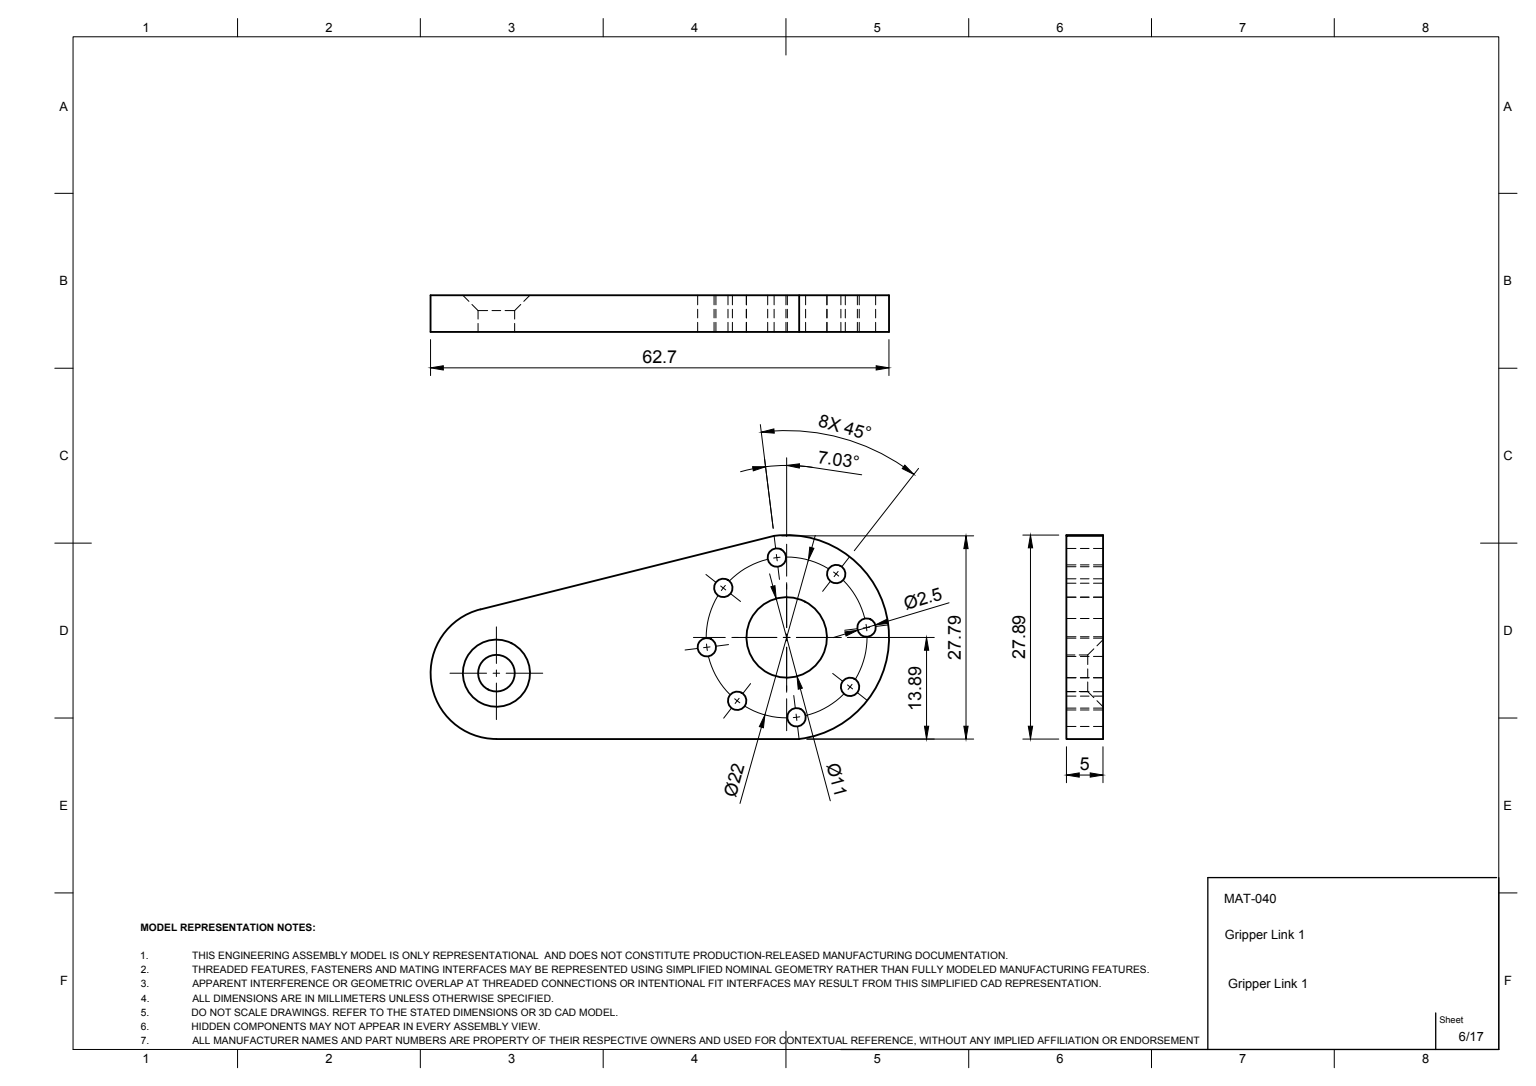
ISO-10303-21;
HEADER;
/* Generated by software containing ST-Developer
 * from STEP Tools, Inc. (www.steptools.com) 
 */

FILE_DESCRIPTION(
/* description */ ('STEP AP214'),
/* implementation_level */ '2;1');

FILE_NAME(
/* name */ 'Gripper Link 1.step',
/* time_stamp */ '2026-11-14T21:53:28-08:00',
/* author */ (''),
/* organization */ (''),
/* preprocessor_version */ 'ST-DEVELOPER v20.2',
/* originating_system */ 'Autodesk Translation Framework v15.17.0.0',
/* authorisation */ '');

FILE_SCHEMA (('AUTOMOTIVE_DESIGN { 1 0 10303 214 3 1 1 }'));
ENDSEC;

DATA;
#10=MECHANICAL_DESIGN_GEOMETRIC_PRESENTATION_REPRESENTATION('',(#329),#20176);
#214=CONICAL_SURFACE('',#11867,4.59,0.785398163397449);
#297=SHAPE_REPRESENTATION_RELATIONSHIP('SRR','None',#20259,#309);
#309=ADVANCED_BREP_SHAPE_REPRESENTATION('',(#356),#20165);
#329=STYLED_ITEM('',(#20337),#356);
#356=MANIFOLD_SOLID_BREP('Body1',#10947);
#516=FACE_BOUND('',#2077,.T.);
#517=FACE_BOUND('',#2078,.T.);
#518=FACE_BOUND('',#2079,.T.);
#519=FACE_BOUND('',#2080,.T.);
#520=FACE_BOUND('',#2081,.T.);
#521=FACE_BOUND('',#2082,.T.);
#522=FACE_BOUND('',#2083,.T.);
#523=FACE_BOUND('',#2084,.T.);
#524=FACE_BOUND('',#2085,.T.);
#525=FACE_BOUND('',#2086,.T.);
#526=FACE_BOUND('',#2088,.T.);
#527=FACE_BOUND('',#2089,.T.);
#528=FACE_BOUND('',#2090,.T.);
#529=FACE_BOUND('',#2091,.T.);
#530=FACE_BOUND('',#2092,.T.);
#531=FACE_BOUND('',#2093,.T.);
#532=FACE_BOUND('',#2094,.T.);
#533=FACE_BOUND('',#2095,.T.);
#534=FACE_BOUND('',#2096,.T.);
#535=FACE_BOUND('',#2097,.T.);
#822=PLANE('',#11900);
#823=PLANE('',#11903);
#824=PLANE('',#11908);
#825=PLANE('',#11909);
#1337=FACE_OUTER_BOUND('',#2065,.T.);
#1338=FACE_OUTER_BOUND('',#2066,.T.);
#1339=FACE_OUTER_BOUND('',#2067,.T.);
#1340=FACE_OUTER_BOUND('',#2068,.T.);
#1341=FACE_OUTER_BOUND('',#2069,.T.);
#1342=FACE_OUTER_BOUND('',#2070,.T.);
#1343=FACE_OUTER_BOUND('',#2071,.T.);
#1344=FACE_OUTER_BOUND('',#2072,.T.);
#1345=FACE_OUTER_BOUND('',#2073,.T.);
#1346=FACE_OUTER_BOUND('',#2074,.T.);
#1347=FACE_OUTER_BOUND('',#2075,.T.);
#1348=FACE_OUTER_BOUND('',#2076,.T.);
#1349=FACE_OUTER_BOUND('',#2087,.T.);
#1350=FACE_OUTER_BOUND('',#2098,.T.);
#1351=FACE_OUTER_BOUND('',#2099,.T.);
#1352=FACE_OUTER_BOUND('',#2100,.T.);
#1353=FACE_OUTER_BOUND('',#2101,.T.);
#2065=EDGE_LOOP('',(#9471,#9472,#9473,#9474,#9475));
#2066=EDGE_LOOP('',(#9476,#9477,#9478,#9479));
#2067=EDGE_LOOP('',(#9480,#9481,#9482,#9483));
#2068=EDGE_LOOP('',(#9484,#9485,#9486,#9487));
#2069=EDGE_LOOP('',(#9488,#9489,#9490,#9491));
#2070=EDGE_LOOP('',(#9492,#9493,#9494,#9495));
#2071=EDGE_LOOP('',(#9496,#9497,#9498,#9499));
#2072=EDGE_LOOP('',(#9500,#9501,#9502,#9503));
#2073=EDGE_LOOP('',(#9504,#9505,#9506,#9507));
#2074=EDGE_LOOP('',(#9508,#9509,#9510,#9511));
#2075=EDGE_LOOP('',(#9512,#9513,#9514,#9515,#9516));
#2076=EDGE_LOOP('',(#9517,#9518,#9519,#9520));
#2077=EDGE_LOOP('',(#9521));
#2078=EDGE_LOOP('',(#9522));
#2079=EDGE_LOOP('',(#9523));
#2080=EDGE_LOOP('',(#9524));
#2081=EDGE_LOOP('',(#9525));
#2082=EDGE_LOOP('',(#9526));
#2083=EDGE_LOOP('',(#9527));
#2084=EDGE_LOOP('',(#9528));
#2085=EDGE_LOOP('',(#9529));
#2086=EDGE_LOOP('',(#9530));
#2087=EDGE_LOOP('',(#9531,#9532,#9533,#9534));
#2088=EDGE_LOOP('',(#9535));
#2089=EDGE_LOOP('',(#9536));
#2090=EDGE_LOOP('',(#9537));
#2091=EDGE_LOOP('',(#9538));
#2092=EDGE_LOOP('',(#9539));
#2093=EDGE_LOOP('',(#9540));
#2094=EDGE_LOOP('',(#9541));
#2095=EDGE_LOOP('',(#9542));
#2096=EDGE_LOOP('',(#9543));
#2097=EDGE_LOOP('',(#9544));
#2098=EDGE_LOOP('',(#9545,#9546,#9547,#9548));
#2099=EDGE_LOOP('',(#9549,#9550,#9551,#9552));
#2100=EDGE_LOOP('',(#9553,#9554,#9555,#9556));
#2101=EDGE_LOOP('',(#9557,#9558,#9559,#9560));
#3069=LINE('',#19370,#4057);
#3070=LINE('',#19377,#4058);
#3071=LINE('',#19383,#4059);
#3072=LINE('',#19389,#4060);
#3073=LINE('',#19395,#4061);
#3074=LINE('',#19401,#4062);
#3075=LINE('',#19407,#4063);
#3076=LINE('',#19413,#4064);
#3077=LINE('',#19419,#4065);
#3078=LINE('',#19425,#4066);
#3079=LINE('',#19429,#4067);
#3080=LINE('',#19434,#4068);
#3081=LINE('',#19438,#4069);
#3082=LINE('',#19445,#4070);
#3083=LINE('',#19448,#4071);
#3084=LINE('',#19450,#4072);
#3085=LINE('',#19451,#4073);
#3086=LINE('',#19453,#4074);
#3087=LINE('',#19454,#4075);
#4057=VECTOR('',#14533,4.59);
#4058=VECTOR('',#14542,1.25);
#4059=VECTOR('',#14549,1.25);
#4060=VECTOR('',#14556,1.25);
#4061=VECTOR('',#14563,1.25);
#4062=VECTOR('',#14570,1.25);
#4063=VECTOR('',#14577,1.25);
#4064=VECTOR('',#14584,1.25);
#4065=VECTOR('',#14591,1.25);
#4066=VECTOR('',#14598,5.5);
#4067=VECTOR('',#14603,2.5);
#4068=VECTOR('',#14608,1000.);
#4069=VECTOR('',#14611,1000.);
#4070=VECTOR('',#14618,1000.);
#4071=VECTOR('',#14621,1000.);
#4072=VECTOR('',#14624,1000.);
#4073=VECTOR('',#14625,1000.);
#4074=VECTOR('',#14628,1000.);
#4075=VECTOR('',#14629,1000.);
#4589=CIRCLE('',#11868,2.5);
#4590=CIRCLE('',#11869,4.59);
#4591=CIRCLE('',#11870,2.5);
#4592=CIRCLE('',#11872,1.25);
#4593=CIRCLE('',#11873,1.25);
#4594=CIRCLE('',#11875,1.25);
#4595=CIRCLE('',#11876,1.25);
#4596=CIRCLE('',#11878,1.25);
#4597=CIRCLE('',#11879,1.25);
#4598=CIRCLE('',#11881,1.25);
#4599=CIRCLE('',#11882,1.25);
#4600=CIRCLE('',#11884,1.25);
#4601=CIRCLE('',#11885,1.25);
#4602=CIRCLE('',#11887,1.25);
#4603=CIRCLE('',#11888,1.25);
#4604=CIRCLE('',#11890,1.25);
#4605=CIRCLE('',#11891,1.25);
#4606=CIRCLE('',#11893,1.25);
#4607=CIRCLE('',#11894,1.25);
#4608=CIRCLE('',#11896,5.5);
#4609=CIRCLE('',#11897,5.5);
#4610=CIRCLE('',#11899,2.5);
#4611=CIRCLE('',#11901,14.);
#4612=CIRCLE('',#11902,9.);
#4613=CIRCLE('',#11904,14.);
#4614=CIRCLE('',#11905,9.);
#5460=VERTEX_POINT('',#19366);
#5461=VERTEX_POINT('',#19367);
#5462=VERTEX_POINT('',#19369);
#5463=VERTEX_POINT('',#19374);
#5464=VERTEX_POINT('',#19376);
#5465=VERTEX_POINT('',#19380);
#5466=VERTEX_POINT('',#19382);
#5467=VERTEX_POINT('',#19386);
#5468=VERTEX_POINT('',#19388);
#5469=VERTEX_POINT('',#19392);
#5470=VERTEX_POINT('',#19394);
#5471=VERTEX_POINT('',#19398);
#5472=VERTEX_POINT('',#19400);
#5473=VERTEX_POINT('',#19404);
#5474=VERTEX_POINT('',#19406);
#5475=VERTEX_POINT('',#19410);
#5476=VERTEX_POINT('',#19412);
#5477=VERTEX_POINT('',#19416);
#5478=VERTEX_POINT('',#19418);
#5479=VERTEX_POINT('',#19422);
#5480=VERTEX_POINT('',#19424);
#5481=VERTEX_POINT('',#19428);
#5482=VERTEX_POINT('',#19432);
#5483=VERTEX_POINT('',#19433);
#5484=VERTEX_POINT('',#19435);
#5485=VERTEX_POINT('',#19437);
#5486=VERTEX_POINT('',#19441);
#5487=VERTEX_POINT('',#19442);
#5488=VERTEX_POINT('',#19444);
#5489=VERTEX_POINT('',#19446);
#6846=EDGE_CURVE('',#5460,#5461,#4589,.T.);
#6847=EDGE_CURVE('',#5461,#5462,#3069,.T.);
#6848=EDGE_CURVE('',#5462,#5462,#4590,.T.);
#6849=EDGE_CURVE('',#5461,#5460,#4591,.T.);
#6850=EDGE_CURVE('',#5463,#5463,#4592,.T.);
#6851=EDGE_CURVE('',#5463,#5464,#3070,.T.);
#6852=EDGE_CURVE('',#5464,#5464,#4593,.T.);
#6853=EDGE_CURVE('',#5465,#5465,#4594,.T.);
#6854=EDGE_CURVE('',#5465,#5466,#3071,.T.);
#6855=EDGE_CURVE('',#5466,#5466,#4595,.T.);
#6856=EDGE_CURVE('',#5467,#5467,#4596,.T.);
#6857=EDGE_CURVE('',#5467,#5468,#3072,.T.);
#6858=EDGE_CURVE('',#5468,#5468,#4597,.T.);
#6859=EDGE_CURVE('',#5469,#5469,#4598,.T.);
#6860=EDGE_CURVE('',#5469,#5470,#3073,.T.);
#6861=EDGE_CURVE('',#5470,#5470,#4599,.T.);
#6862=EDGE_CURVE('',#5471,#5471,#4600,.T.);
#6863=EDGE_CURVE('',#5471,#5472,#3074,.T.);
#6864=EDGE_CURVE('',#5472,#5472,#4601,.T.);
#6865=EDGE_CURVE('',#5473,#5473,#4602,.T.);
#6866=EDGE_CURVE('',#5473,#5474,#3075,.T.);
#6867=EDGE_CURVE('',#5474,#5474,#4603,.T.);
#6868=EDGE_CURVE('',#5475,#5475,#4604,.T.);
#6869=EDGE_CURVE('',#5475,#5476,#3076,.T.);
#6870=EDGE_CURVE('',#5476,#5476,#4605,.T.);
#6871=EDGE_CURVE('',#5477,#5477,#4606,.T.);
#6872=EDGE_CURVE('',#5477,#5478,#3077,.T.);
#6873=EDGE_CURVE('',#5478,#5478,#4607,.T.);
#6874=EDGE_CURVE('',#5479,#5479,#4608,.T.);
#6875=EDGE_CURVE('',#5479,#5480,#3078,.T.);
#6876=EDGE_CURVE('',#5480,#5480,#4609,.T.);
#6877=EDGE_CURVE('',#5460,#5481,#3079,.T.);
#6878=EDGE_CURVE('',#5481,#5481,#4610,.T.);
#6879=EDGE_CURVE('',#5482,#5483,#3080,.T.);
#6880=EDGE_CURVE('',#5482,#5484,#4611,.T.);
#6881=EDGE_CURVE('',#5484,#5485,#3081,.T.);
#6882=EDGE_CURVE('',#5485,#5483,#4612,.T.);
#6883=EDGE_CURVE('',#5486,#5487,#4613,.T.);
#6884=EDGE_CURVE('',#5486,#5488,#3082,.T.);
#6885=EDGE_CURVE('',#5489,#5488,#4614,.T.);
#6886=EDGE_CURVE('',#5487,#5489,#3083,.T.);
#6887=EDGE_CURVE('',#5484,#5487,#3084,.T.);
#6888=EDGE_CURVE('',#5482,#5486,#3085,.T.);
#6889=EDGE_CURVE('',#5489,#5485,#3086,.T.);
#6890=EDGE_CURVE('',#5488,#5483,#3087,.T.);
#9471=ORIENTED_EDGE('',*,*,#6846,.T.);
#9472=ORIENTED_EDGE('',*,*,#6847,.T.);
#9473=ORIENTED_EDGE('',*,*,#6848,.T.);
#9474=ORIENTED_EDGE('',*,*,#6847,.F.);
#9475=ORIENTED_EDGE('',*,*,#6849,.T.);
#9476=ORIENTED_EDGE('',*,*,#6850,.F.);
#9477=ORIENTED_EDGE('',*,*,#6851,.T.);
#9478=ORIENTED_EDGE('',*,*,#6852,.T.);
#9479=ORIENTED_EDGE('',*,*,#6851,.F.);
#9480=ORIENTED_EDGE('',*,*,#6853,.F.);
#9481=ORIENTED_EDGE('',*,*,#6854,.T.);
#9482=ORIENTED_EDGE('',*,*,#6855,.T.);
#9483=ORIENTED_EDGE('',*,*,#6854,.F.);
#9484=ORIENTED_EDGE('',*,*,#6856,.F.);
#9485=ORIENTED_EDGE('',*,*,#6857,.T.);
#9486=ORIENTED_EDGE('',*,*,#6858,.T.);
#9487=ORIENTED_EDGE('',*,*,#6857,.F.);
#9488=ORIENTED_EDGE('',*,*,#6859,.F.);
#9489=ORIENTED_EDGE('',*,*,#6860,.T.);
#9490=ORIENTED_EDGE('',*,*,#6861,.T.);
#9491=ORIENTED_EDGE('',*,*,#6860,.F.);
#9492=ORIENTED_EDGE('',*,*,#6862,.F.);
#9493=ORIENTED_EDGE('',*,*,#6863,.T.);
#9494=ORIENTED_EDGE('',*,*,#6864,.T.);
#9495=ORIENTED_EDGE('',*,*,#6863,.F.);
#9496=ORIENTED_EDGE('',*,*,#6865,.F.);
#9497=ORIENTED_EDGE('',*,*,#6866,.T.);
#9498=ORIENTED_EDGE('',*,*,#6867,.T.);
#9499=ORIENTED_EDGE('',*,*,#6866,.F.);
#9500=ORIENTED_EDGE('',*,*,#6868,.F.);
#9501=ORIENTED_EDGE('',*,*,#6869,.T.);
#9502=ORIENTED_EDGE('',*,*,#6870,.T.);
#9503=ORIENTED_EDGE('',*,*,#6869,.F.);
#9504=ORIENTED_EDGE('',*,*,#6871,.F.);
#9505=ORIENTED_EDGE('',*,*,#6872,.T.);
#9506=ORIENTED_EDGE('',*,*,#6873,.T.);
#9507=ORIENTED_EDGE('',*,*,#6872,.F.);
#9508=ORIENTED_EDGE('',*,*,#6874,.T.);
#9509=ORIENTED_EDGE('',*,*,#6875,.T.);
#9510=ORIENTED_EDGE('',*,*,#6876,.F.);
#9511=ORIENTED_EDGE('',*,*,#6875,.F.);
#9512=ORIENTED_EDGE('',*,*,#6846,.F.);
#9513=ORIENTED_EDGE('',*,*,#6877,.T.);
#9514=ORIENTED_EDGE('',*,*,#6878,.F.);
#9515=ORIENTED_EDGE('',*,*,#6877,.F.);
#9516=ORIENTED_EDGE('',*,*,#6849,.F.);
#9517=ORIENTED_EDGE('',*,*,#6879,.F.);
#9518=ORIENTED_EDGE('',*,*,#6880,.T.);
#9519=ORIENTED_EDGE('',*,*,#6881,.T.);
#9520=ORIENTED_EDGE('',*,*,#6882,.T.);
#9521=ORIENTED_EDGE('',*,*,#6852,.F.);
#9522=ORIENTED_EDGE('',*,*,#6855,.F.);
#9523=ORIENTED_EDGE('',*,*,#6858,.F.);
#9524=ORIENTED_EDGE('',*,*,#6861,.F.);
#9525=ORIENTED_EDGE('',*,*,#6864,.F.);
#9526=ORIENTED_EDGE('',*,*,#6867,.F.);
#9527=ORIENTED_EDGE('',*,*,#6870,.F.);
#9528=ORIENTED_EDGE('',*,*,#6873,.F.);
#9529=ORIENTED_EDGE('',*,*,#6874,.F.);
#9530=ORIENTED_EDGE('',*,*,#6848,.F.);
#9531=ORIENTED_EDGE('',*,*,#6883,.F.);
#9532=ORIENTED_EDGE('',*,*,#6884,.T.);
#9533=ORIENTED_EDGE('',*,*,#6885,.F.);
#9534=ORIENTED_EDGE('',*,*,#6886,.F.);
#9535=ORIENTED_EDGE('',*,*,#6876,.T.);
#9536=ORIENTED_EDGE('',*,*,#6850,.T.);
#9537=ORIENTED_EDGE('',*,*,#6853,.T.);
#9538=ORIENTED_EDGE('',*,*,#6856,.T.);
#9539=ORIENTED_EDGE('',*,*,#6859,.T.);
#9540=ORIENTED_EDGE('',*,*,#6862,.T.);
#9541=ORIENTED_EDGE('',*,*,#6865,.T.);
#9542=ORIENTED_EDGE('',*,*,#6868,.T.);
#9543=ORIENTED_EDGE('',*,*,#6871,.T.);
#9544=ORIENTED_EDGE('',*,*,#6878,.T.);
#9545=ORIENTED_EDGE('',*,*,#6883,.T.);
#9546=ORIENTED_EDGE('',*,*,#6887,.F.);
#9547=ORIENTED_EDGE('',*,*,#6880,.F.);
#9548=ORIENTED_EDGE('',*,*,#6888,.T.);
#9549=ORIENTED_EDGE('',*,*,#6882,.F.);
#9550=ORIENTED_EDGE('',*,*,#6889,.F.);
#9551=ORIENTED_EDGE('',*,*,#6885,.T.);
#9552=ORIENTED_EDGE('',*,*,#6890,.T.);
#9553=ORIENTED_EDGE('',*,*,#6879,.T.);
#9554=ORIENTED_EDGE('',*,*,#6890,.F.);
#9555=ORIENTED_EDGE('',*,*,#6884,.F.);
#9556=ORIENTED_EDGE('',*,*,#6888,.F.);
#9557=ORIENTED_EDGE('',*,*,#6881,.F.);
#9558=ORIENTED_EDGE('',*,*,#6887,.T.);
#9559=ORIENTED_EDGE('',*,*,#6886,.T.);
#9560=ORIENTED_EDGE('',*,*,#6889,.T.);
#10299=CYLINDRICAL_SURFACE('',#11871,1.25);
#10300=CYLINDRICAL_SURFACE('',#11874,1.25);
#10301=CYLINDRICAL_SURFACE('',#11877,1.25);
#10302=CYLINDRICAL_SURFACE('',#11880,1.25);
#10303=CYLINDRICAL_SURFACE('',#11883,1.25);
#10304=CYLINDRICAL_SURFACE('',#11886,1.25);
#10305=CYLINDRICAL_SURFACE('',#11889,1.25);
#10306=CYLINDRICAL_SURFACE('',#11892,1.25);
#10307=CYLINDRICAL_SURFACE('',#11895,5.5);
#10308=CYLINDRICAL_SURFACE('',#11898,2.5);
#10309=CYLINDRICAL_SURFACE('',#11906,14.);
#10310=CYLINDRICAL_SURFACE('',#11907,9.);
#10789=ADVANCED_FACE('',(#1337),#214,.F.);
#10790=ADVANCED_FACE('',(#1338),#10299,.F.);
#10791=ADVANCED_FACE('',(#1339),#10300,.F.);
#10792=ADVANCED_FACE('',(#1340),#10301,.F.);
#10793=ADVANCED_FACE('',(#1341),#10302,.F.);
#10794=ADVANCED_FACE('',(#1342),#10303,.F.);
#10795=ADVANCED_FACE('',(#1343),#10304,.F.);
#10796=ADVANCED_FACE('',(#1344),#10305,.F.);
#10797=ADVANCED_FACE('',(#1345),#10306,.F.);
#10798=ADVANCED_FACE('',(#1346),#10307,.F.);
#10799=ADVANCED_FACE('',(#1347),#10308,.F.);
#10800=ADVANCED_FACE('',(#1348,#516,#517,#518,#519,#520,#521,#522,#523,
#524,#525),#822,.T.);
#10801=ADVANCED_FACE('',(#1349,#526,#527,#528,#529,#530,#531,#532,#533,
#534,#535),#823,.F.);
#10802=ADVANCED_FACE('',(#1350),#10309,.T.);
#10803=ADVANCED_FACE('',(#1351),#10310,.T.);
#10804=ADVANCED_FACE('',(#1352),#824,.F.);
#10805=ADVANCED_FACE('',(#1353),#825,.T.);
#10947=CLOSED_SHELL('',(#10789,#10790,#10791,#10792,#10793,#10794,#10795,
#10796,#10797,#10798,#10799,#10800,#10801,#10802,#10803,#10804,#10805));
#11866=AXIS2_PLACEMENT_3D('',#19364,#14527,#14528);
#11867=AXIS2_PLACEMENT_3D('',#19365,#14529,#14530);
#11868=AXIS2_PLACEMENT_3D('',#19368,#14531,#14532);
#11869=AXIS2_PLACEMENT_3D('',#19371,#14534,#14535);
#11870=AXIS2_PLACEMENT_3D('',#19372,#14536,#14537);
#11871=AXIS2_PLACEMENT_3D('',#19373,#14538,#14539);
#11872=AXIS2_PLACEMENT_3D('',#19375,#14540,#14541);
#11873=AXIS2_PLACEMENT_3D('',#19378,#14543,#14544);
#11874=AXIS2_PLACEMENT_3D('',#19379,#14545,#14546);
#11875=AXIS2_PLACEMENT_3D('',#19381,#14547,#14548);
#11876=AXIS2_PLACEMENT_3D('',#19384,#14550,#14551);
#11877=AXIS2_PLACEMENT_3D('',#19385,#14552,#14553);
#11878=AXIS2_PLACEMENT_3D('',#19387,#14554,#14555);
#11879=AXIS2_PLACEMENT_3D('',#19390,#14557,#14558);
#11880=AXIS2_PLACEMENT_3D('',#19391,#14559,#14560);
#11881=AXIS2_PLACEMENT_3D('',#19393,#14561,#14562);
#11882=AXIS2_PLACEMENT_3D('',#19396,#14564,#14565);
#11883=AXIS2_PLACEMENT_3D('',#19397,#14566,#14567);
#11884=AXIS2_PLACEMENT_3D('',#19399,#14568,#14569);
#11885=AXIS2_PLACEMENT_3D('',#19402,#14571,#14572);
#11886=AXIS2_PLACEMENT_3D('',#19403,#14573,#14574);
#11887=AXIS2_PLACEMENT_3D('',#19405,#14575,#14576);
#11888=AXIS2_PLACEMENT_3D('',#19408,#14578,#14579);
#11889=AXIS2_PLACEMENT_3D('',#19409,#14580,#14581);
#11890=AXIS2_PLACEMENT_3D('',#19411,#14582,#14583);
#11891=AXIS2_PLACEMENT_3D('',#19414,#14585,#14586);
#11892=AXIS2_PLACEMENT_3D('',#19415,#14587,#14588);
#11893=AXIS2_PLACEMENT_3D('',#19417,#14589,#14590);
#11894=AXIS2_PLACEMENT_3D('',#19420,#14592,#14593);
#11895=AXIS2_PLACEMENT_3D('',#19421,#14594,#14595);
#11896=AXIS2_PLACEMENT_3D('',#19423,#14596,#14597);
#11897=AXIS2_PLACEMENT_3D('',#19426,#14599,#14600);
#11898=AXIS2_PLACEMENT_3D('',#19427,#14601,#14602);
#11899=AXIS2_PLACEMENT_3D('',#19430,#14604,#14605);
#11900=AXIS2_PLACEMENT_3D('',#19431,#14606,#14607);
#11901=AXIS2_PLACEMENT_3D('',#19436,#14609,#14610);
#11902=AXIS2_PLACEMENT_3D('',#19439,#14612,#14613);
#11903=AXIS2_PLACEMENT_3D('',#19440,#14614,#14615);
#11904=AXIS2_PLACEMENT_3D('',#19443,#14616,#14617);
#11905=AXIS2_PLACEMENT_3D('',#19447,#14619,#14620);
#11906=AXIS2_PLACEMENT_3D('',#19449,#14622,#14623);
#11907=AXIS2_PLACEMENT_3D('',#19452,#14626,#14627);
#11908=AXIS2_PLACEMENT_3D('',#19455,#14630,#14631);
#11909=AXIS2_PLACEMENT_3D('',#19456,#14632,#14633);
#14527=DIRECTION('axis',(0.,0.,1.));
#14528=DIRECTION('refdir',(1.,0.,0.));
#14529=DIRECTION('center_axis',(0.,1.,0.));
#14530=DIRECTION('ref_axis',(0.,0.,1.));
#14531=DIRECTION('center_axis',(0.,-1.,0.));
#14532=DIRECTION('ref_axis',(0.,0.,1.));
#14533=DIRECTION('',(-8.65956056235494E-17,0.707106781186547,-0.707106781186548));
#14534=DIRECTION('center_axis',(0.,1.,0.));
#14535=DIRECTION('ref_axis',(0.,0.,1.));
#14536=DIRECTION('center_axis',(0.,-1.,0.));
#14537=DIRECTION('ref_axis',(0.,0.,1.));
#14538=DIRECTION('center_axis',(0.,1.,0.));
#14539=DIRECTION('ref_axis',(0.,0.,1.));
#14540=DIRECTION('center_axis',(0.,1.,0.));
#14541=DIRECTION('ref_axis',(0.,0.,1.));
#14542=DIRECTION('',(0.,1.,0.));
#14543=DIRECTION('center_axis',(0.,1.,0.));
#14544=DIRECTION('ref_axis',(0.,0.,1.));
#14545=DIRECTION('center_axis',(0.,1.,0.));
#14546=DIRECTION('ref_axis',(0.,0.,1.));
#14547=DIRECTION('center_axis',(0.,1.,0.));
#14548=DIRECTION('ref_axis',(0.,0.,1.));
#14549=DIRECTION('',(0.,1.,0.));
#14550=DIRECTION('center_axis',(0.,1.,0.));
#14551=DIRECTION('ref_axis',(0.,0.,1.));
#14552=DIRECTION('center_axis',(0.,1.,0.));
#14553=DIRECTION('ref_axis',(0.,0.,1.));
#14554=DIRECTION('center_axis',(0.,1.,0.));
#14555=DIRECTION('ref_axis',(0.,0.,1.));
#14556=DIRECTION('',(0.,1.,0.));
#14557=DIRECTION('center_axis',(0.,1.,0.));
#14558=DIRECTION('ref_axis',(0.,0.,1.));
#14559=DIRECTION('center_axis',(0.,1.,0.));
#14560=DIRECTION('ref_axis',(0.,0.,1.));
#14561=DIRECTION('center_axis',(0.,1.,0.));
#14562=DIRECTION('ref_axis',(0.,0.,1.));
#14563=DIRECTION('',(0.,1.,0.));
#14564=DIRECTION('center_axis',(0.,1.,0.));
#14565=DIRECTION('ref_axis',(0.,0.,1.));
#14566=DIRECTION('center_axis',(0.,1.,0.));
#14567=DIRECTION('ref_axis',(0.,0.,1.));
#14568=DIRECTION('center_axis',(0.,1.,0.));
#14569=DIRECTION('ref_axis',(0.,0.,1.));
#14570=DIRECTION('',(0.,1.,0.));
#14571=DIRECTION('center_axis',(0.,1.,0.));
#14572=DIRECTION('ref_axis',(0.,0.,1.));
#14573=DIRECTION('center_axis',(0.,1.,0.));
#14574=DIRECTION('ref_axis',(0.,0.,1.));
#14575=DIRECTION('center_axis',(0.,1.,0.));
#14576=DIRECTION('ref_axis',(0.,0.,1.));
#14577=DIRECTION('',(0.,1.,0.));
#14578=DIRECTION('center_axis',(0.,1.,0.));
#14579=DIRECTION('ref_axis',(0.,0.,1.));
#14580=DIRECTION('center_axis',(0.,1.,0.));
#14581=DIRECTION('ref_axis',(0.,0.,1.));
#14582=DIRECTION('center_axis',(0.,1.,0.));
#14583=DIRECTION('ref_axis',(0.,0.,1.));
#14584=DIRECTION('',(0.,1.,0.));
#14585=DIRECTION('center_axis',(0.,1.,0.));
#14586=DIRECTION('ref_axis',(0.,0.,1.));
#14587=DIRECTION('center_axis',(0.,1.,0.));
#14588=DIRECTION('ref_axis',(0.,0.,1.));
#14589=DIRECTION('center_axis',(0.,1.,0.));
#14590=DIRECTION('ref_axis',(0.,0.,1.));
#14591=DIRECTION('',(0.,1.,0.));
#14592=DIRECTION('center_axis',(0.,1.,0.));
#14593=DIRECTION('ref_axis',(0.,0.,1.));
#14594=DIRECTION('center_axis',(0.,-1.,0.));
#14595=DIRECTION('ref_axis',(0.,0.,-1.));
#14596=DIRECTION('center_axis',(0.,1.,0.));
#14597=DIRECTION('ref_axis',(0.,0.,1.));
#14598=DIRECTION('',(0.,-1.,0.));
#14599=DIRECTION('center_axis',(0.,1.,0.));
#14600=DIRECTION('ref_axis',(0.,0.,1.));
#14601=DIRECTION('center_axis',(0.,-1.,0.));
#14602=DIRECTION('ref_axis',(0.,0.,-1.));
#14603=DIRECTION('',(0.,-1.,0.));
#14604=DIRECTION('center_axis',(0.,1.,0.));
#14605=DIRECTION('ref_axis',(0.,0.,1.));
#14606=DIRECTION('center_axis',(0.,1.,0.));
#14607=DIRECTION('ref_axis',(0.,0.,1.));
#14608=DIRECTION('',(0.122369609545525,0.,-0.992484598701499));
#14609=DIRECTION('center_axis',(0.,1.,0.));
#14610=DIRECTION('ref_axis',(0.,0.,1.));
#14611=DIRECTION('',(-0.122369609545525,0.,-0.992484598701499));
#14612=DIRECTION('center_axis',(0.,1.,0.));
#14613=DIRECTION('ref_axis',(0.,0.,1.));
#14614=DIRECTION('center_axis',(0.,1.,0.));
#14615=DIRECTION('ref_axis',(0.,0.,1.));
#14616=DIRECTION('center_axis',(0.,1.,0.));
#14617=DIRECTION('ref_axis',(0.,0.,1.));
#14618=DIRECTION('',(0.122369609545525,0.,-0.992484598701499));
#14619=DIRECTION('center_axis',(0.,1.,0.));
#14620=DIRECTION('ref_axis',(0.,0.,1.));
#14621=DIRECTION('',(-0.122369609545525,0.,-0.992484598701499));
#14622=DIRECTION('center_axis',(0.,-1.,0.));
#14623=DIRECTION('ref_axis',(1.22464679914735E-16,0.,1.));
#14624=DIRECTION('',(0.,-1.,0.));
#14625=DIRECTION('',(0.,-1.,0.));
#14626=DIRECTION('center_axis',(0.,1.,0.));
#14627=DIRECTION('ref_axis',(1.22464679914735E-16,0.,-1.));
#14628=DIRECTION('',(0.,1.,0.));
#14629=DIRECTION('',(0.,1.,0.));
#14630=DIRECTION('center_axis',(0.992484598701499,0.,0.122369609545525));
#14631=DIRECTION('ref_axis',(0.122369609545525,0.,-0.992484598701499));
#14632=DIRECTION('center_axis',(0.992484598701499,0.,-0.122369609545525));
#14633=DIRECTION('ref_axis',(-0.122369609545525,0.,-0.992484598701499));
#19364=CARTESIAN_POINT('',(0.,0.,0.));
#19365=CARTESIAN_POINT('Origin',(0.,5.,-40.));
#19366=CARTESIAN_POINT('',(3.06161699786838E-16,2.91,-37.5));
#19367=CARTESIAN_POINT('',(-3.06161699786838E-16,2.91,-42.5));
#19368=CARTESIAN_POINT('Origin',(0.,2.91,-40.));
#19369=CARTESIAN_POINT('',(-5.62112880808636E-16,5.,-44.59));
#19370=CARTESIAN_POINT('',(-5.62112880808636E-16,5.,-44.59));
#19371=CARTESIAN_POINT('Origin',(0.,5.,-40.));
#19372=CARTESIAN_POINT('Origin',(0.,2.91,-40.));
#19373=CARTESIAN_POINT('Origin',(-7.77817459305202,0.,-7.77817459305202));
#19374=CARTESIAN_POINT('',(-7.77817459305202,0.,-9.02817459305202));
#19375=CARTESIAN_POINT('Origin',(-7.77817459305202,0.,-7.77817459305202));
#19376=CARTESIAN_POINT('',(-7.77817459305202,5.,-9.02817459305202));
#19377=CARTESIAN_POINT('',(-7.77817459305202,0.,-9.02817459305202));
#19378=CARTESIAN_POINT('Origin',(-7.77817459305202,5.,-7.77817459305202));
#19379=CARTESIAN_POINT('Origin',(-11.,0.,2.05998412772246E-15));
#19380=CARTESIAN_POINT('',(-11.,0.,-1.25));
#19381=CARTESIAN_POINT('Origin',(-11.,0.,2.05998412772246E-15));
#19382=CARTESIAN_POINT('',(-11.,5.,-1.25));
#19383=CARTESIAN_POINT('',(-11.,0.,-1.25));
#19384=CARTESIAN_POINT('Origin',(-11.,5.,2.05998412772246E-15));
#19385=CARTESIAN_POINT('Origin',(-7.77817459305202,0.,7.77817459305202));
#19386=CARTESIAN_POINT('',(-7.77817459305202,0.,6.52817459305202));
#19387=CARTESIAN_POINT('Origin',(-7.77817459305202,0.,7.77817459305202));
#19388=CARTESIAN_POINT('',(-7.77817459305202,5.,6.52817459305202));
#19389=CARTESIAN_POINT('',(-7.77817459305202,0.,6.52817459305202));
#19390=CARTESIAN_POINT('Origin',(-7.77817459305202,5.,7.77817459305202));
#19391=CARTESIAN_POINT('Origin',(1.30104260698261E-15,0.,11.));
#19392=CARTESIAN_POINT('',(1.14796175708919E-15,0.,9.75));
#19393=CARTESIAN_POINT('Origin',(1.30104260698261E-15,0.,11.));
#19394=CARTESIAN_POINT('',(1.14796175708919E-15,5.,9.75));
#19395=CARTESIAN_POINT('',(1.14796175708919E-15,0.,9.75));
#19396=CARTESIAN_POINT('Origin',(1.30104260698261E-15,5.,11.));
#19397=CARTESIAN_POINT('Origin',(7.77817459305202,0.,7.77817459305202));
#19398=CARTESIAN_POINT('',(7.77817459305202,0.,6.52817459305202));
#19399=CARTESIAN_POINT('Origin',(7.77817459305202,0.,7.77817459305202));
#19400=CARTESIAN_POINT('',(7.77817459305202,5.,6.52817459305202));
#19401=CARTESIAN_POINT('',(7.77817459305202,0.,6.52817459305202));
#19402=CARTESIAN_POINT('Origin',(7.77817459305202,5.,7.77817459305202));
#19403=CARTESIAN_POINT('Origin',(11.,0.,-8.67361737988404E-16));
#19404=CARTESIAN_POINT('',(11.,0.,-1.25));
#19405=CARTESIAN_POINT('Origin',(11.,0.,-8.67361737988404E-16));
#19406=CARTESIAN_POINT('',(11.,5.,-1.25));
#19407=CARTESIAN_POINT('',(11.,0.,-1.25));
#19408=CARTESIAN_POINT('Origin',(11.,5.,-8.67361737988404E-16));
#19409=CARTESIAN_POINT('Origin',(7.77817459305202,0.,-7.77817459305202));
#19410=CARTESIAN_POINT('',(7.77817459305202,0.,-9.02817459305203));
#19411=CARTESIAN_POINT('Origin',(7.77817459305202,0.,-7.77817459305202));
#19412=CARTESIAN_POINT('',(7.77817459305202,5.,-9.02817459305203));
#19413=CARTESIAN_POINT('',(7.77817459305202,0.,-9.02817459305203));
#19414=CARTESIAN_POINT('Origin',(7.77817459305202,5.,-7.77817459305202));
#19415=CARTESIAN_POINT('Origin',(0.,0.,-11.));
#19416=CARTESIAN_POINT('',(-1.53080849893419E-16,0.,-12.25));
#19417=CARTESIAN_POINT('Origin',(0.,0.,-11.));
#19418=CARTESIAN_POINT('',(-1.53080849893419E-16,5.,-12.25));
#19419=CARTESIAN_POINT('',(-1.53080849893419E-16,0.,-12.25));
#19420=CARTESIAN_POINT('Origin',(0.,5.,-11.));
#19421=CARTESIAN_POINT('Origin',(0.,5.,0.));
#19422=CARTESIAN_POINT('',(-6.73555739531044E-16,5.,5.5));
#19423=CARTESIAN_POINT('Origin',(0.,5.,0.));
#19424=CARTESIAN_POINT('',(-6.73555739531044E-16,0.,5.5));
#19425=CARTESIAN_POINT('',(-6.73555739531044E-16,5.,5.5));
#19426=CARTESIAN_POINT('Origin',(0.,0.,0.));
#19427=CARTESIAN_POINT('Origin',(0.,5.,-40.));
#19428=CARTESIAN_POINT('',(-3.06161699786839E-16,0.,-37.5));
#19429=CARTESIAN_POINT('',(-3.06161699786839E-16,5.,-37.5));
#19430=CARTESIAN_POINT('Origin',(0.,0.,-40.));
#19431=CARTESIAN_POINT('Origin',(0.,5.,0.));
#19432=CARTESIAN_POINT('',(-14.,5.,0.));
#19433=CARTESIAN_POINT('',(-8.9323613883135,5.,-41.1013264859097));
#19434=CARTESIAN_POINT('',(-13.7903595012355,5.,-1.70029933952269));
#19435=CARTESIAN_POINT('',(14.,5.,0.));
#19436=CARTESIAN_POINT('Origin',(0.,5.,0.));
#19437=CARTESIAN_POINT('',(8.9323613883135,5.,-41.1013264859097));
#19438=CARTESIAN_POINT('',(13.7903595012355,5.,-1.70029933952269));
#19439=CARTESIAN_POINT('Origin',(0.,5.,-40.));
#19440=CARTESIAN_POINT('Origin',(0.,0.,0.));
#19441=CARTESIAN_POINT('',(-14.,0.,0.));
#19442=CARTESIAN_POINT('',(14.,0.,0.));
#19443=CARTESIAN_POINT('Origin',(0.,0.,0.));
#19444=CARTESIAN_POINT('',(-8.9323613883135,0.,-41.1013264859097));
#19445=CARTESIAN_POINT('',(-13.7903595012355,0.,-1.70029933952269));
#19446=CARTESIAN_POINT('',(8.9323613883135,0.,-41.1013264859097));
#19447=CARTESIAN_POINT('Origin',(0.,0.,-40.));
#19448=CARTESIAN_POINT('',(13.7903595012355,0.,-1.70029933952269));
#19449=CARTESIAN_POINT('Origin',(0.,5.,0.));
#19450=CARTESIAN_POINT('',(14.,5.,0.));
#19451=CARTESIAN_POINT('',(-14.,5.,0.));
#19452=CARTESIAN_POINT('Origin',(0.,0.,-40.));
#19453=CARTESIAN_POINT('',(8.9323613883135,0.,-41.1013264859097));
#19454=CARTESIAN_POINT('',(-8.9323613883135,0.,-41.1013264859097));
#19455=CARTESIAN_POINT('Origin',(-13.7903595012355,0.,-1.70029933952269));
#19456=CARTESIAN_POINT('Origin',(13.7903595012355,0.,-1.70029933952269));
#20149=UNCERTAINTY_MEASURE_WITH_UNIT(LENGTH_MEASURE(0.01),#20177,
'DISTANCE_ACCURACY_VALUE',
'Maximum model space distance between geometric entities at asserted c
onnectivities');
#20160=UNCERTAINTY_MEASURE_WITH_UNIT(LENGTH_MEASURE(0.01),#20177,
'DISTANCE_ACCURACY_VALUE',
'Maximum model space distance between geometric entities at asserted c
onnectivities');
#20165=(
GEOMETRIC_REPRESENTATION_CONTEXT(3)
GLOBAL_UNCERTAINTY_ASSIGNED_CONTEXT((#20149))
GLOBAL_UNIT_ASSIGNED_CONTEXT((#20177,#20179,#20180))
REPRESENTATION_CONTEXT('','3D')
);
#20176=(
GEOMETRIC_REPRESENTATION_CONTEXT(3)
GLOBAL_UNCERTAINTY_ASSIGNED_CONTEXT((#20160))
GLOBAL_UNIT_ASSIGNED_CONTEXT((#20177,#20179,#20180))
REPRESENTATION_CONTEXT('','3D')
);
#20177=(
LENGTH_UNIT()
NAMED_UNIT(*)
SI_UNIT(.MILLI.,.METRE.)
);
#20179=(
NAMED_UNIT(*)
PLANE_ANGLE_UNIT()
SI_UNIT($,.RADIAN.)
);
#20180=(
NAMED_UNIT(*)
SI_UNIT($,.STERADIAN.)
SOLID_ANGLE_UNIT()
);
#20185=SHAPE_DEFINITION_REPRESENTATION(#20200,#20259);
#20200=PRODUCT_DEFINITION_SHAPE('',$,#20275);
#20259=SHAPE_REPRESENTATION('',(#11866),#20165);
#20270=PRODUCT_DEFINITION_CONTEXT('part definition',#20317,'design');
#20275=PRODUCT_DEFINITION('Gripper Link 1','Gripper Link 1',#20290,#20270);
#20290=PRODUCT_DEFINITION_FORMATION('',$,#20323);
#20317=APPLICATION_CONTEXT(
'Core Data for Automotive Mechanical Design Process');
#20318=PRODUCT_CONTEXT('part definition',#20317,'mechanical');
#20323=PRODUCT('Gripper Link 1','Gripper Link 1',$,(#20318));
#20337=PRESENTATION_STYLE_ASSIGNMENT((#20342));
#20342=SURFACE_STYLE_USAGE(.BOTH.,#20347);
#20347=SURFACE_SIDE_STYLE('',(#20352));
#20352=SURFACE_STYLE_FILL_AREA(#20357);
#20357=FILL_AREA_STYLE('Opaque(31,36,43)',(#20362));
#20362=FILL_AREA_STYLE_COLOUR('Opaque(31,36,43)',#20367);
#20367=COLOUR_RGB('Opaque(31,36,43)',0.12156862745098,0.141176470588235,
0.168627450980392);
ENDSEC;
END-ISO-10303-21;
